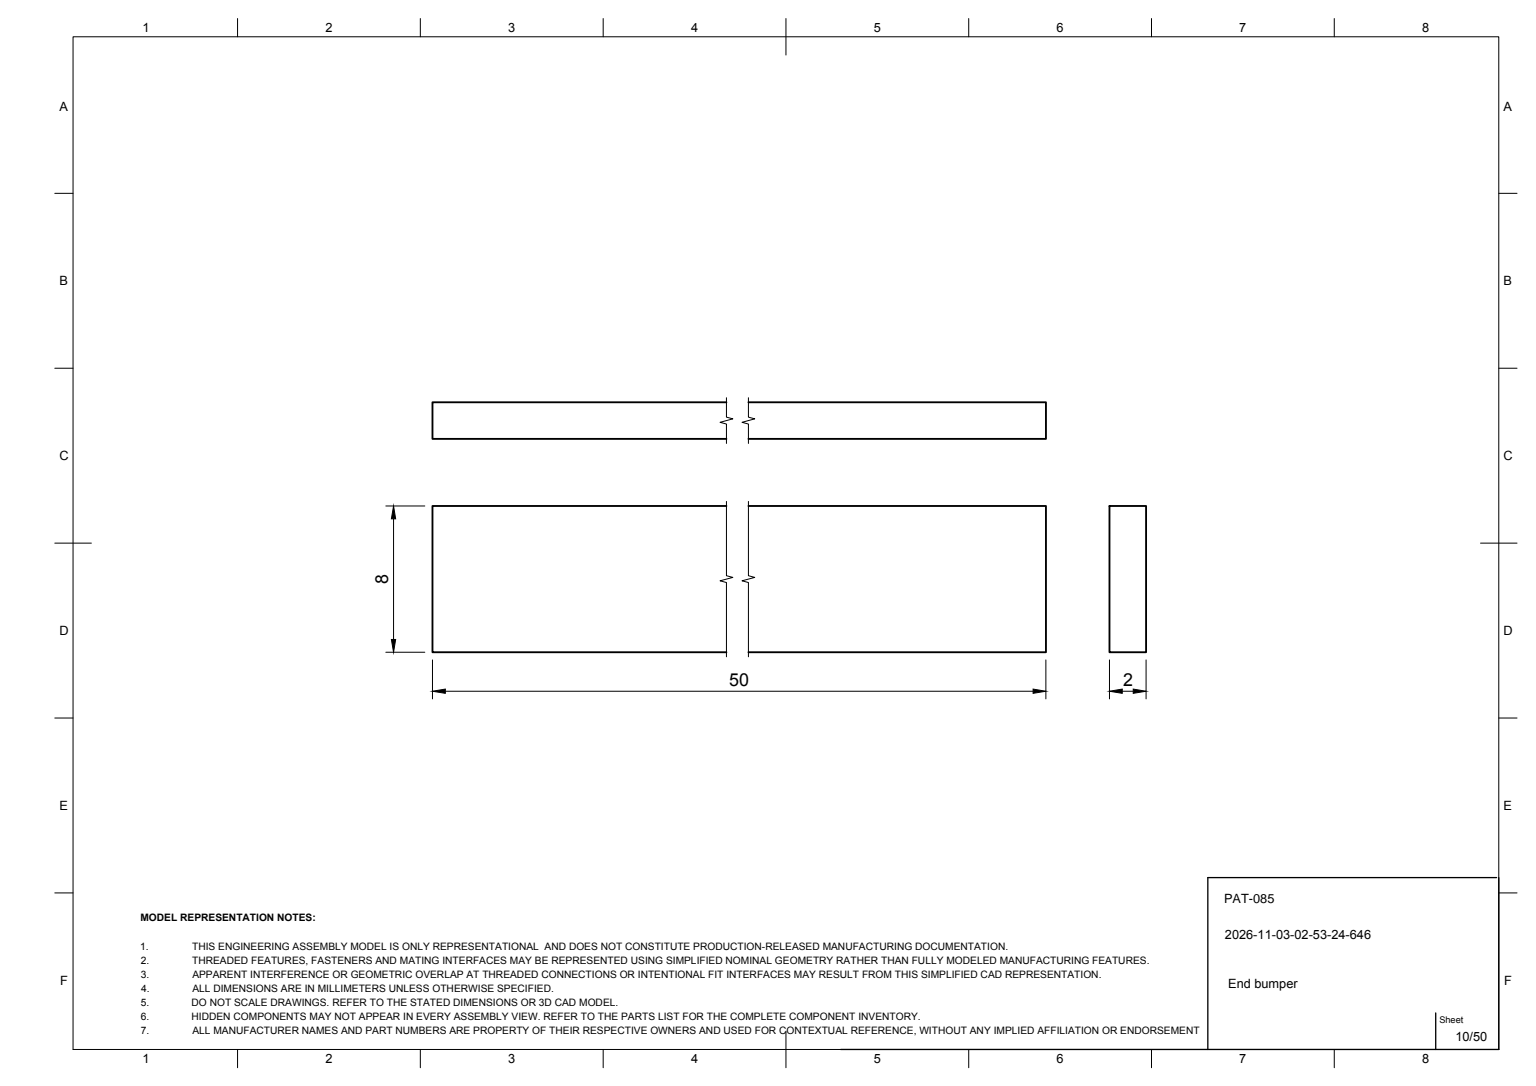
ISO-10303-21;
HEADER;
/* Generated by software containing ST-Developer
 * from STEP Tools, Inc. (www.steptools.com) 
 */

FILE_DESCRIPTION(
/* description */ ('Rack and pinion manual slide'),
/* implementation_level */ '2;1');

FILE_NAME(
/* name */ 'End bumper.step',
/* time_stamp */ '2026-10-28T03:22:49-07:00',
/* author */ (''),
/* organization */ (''),
/* preprocessor_version */ 'ST-DEVELOPER v20.2',
/* originating_system */ 'Autodesk Translation Framework v15.17.0.0',
/* authorisation */ '');

FILE_SCHEMA (('AUTOMOTIVE_DESIGN { 1 0 10303 214 3 1 1 }'));
ENDSEC;

DATA;
#10=MECHANICAL_DESIGN_GEOMETRIC_PRESENTATION_REPRESENTATION('',(#737),#34851);
#645=SHAPE_REPRESENTATION_RELATIONSHIP('SRR','None',#35080,#691);
#691=ADVANCED_BREP_SHAPE_REPRESENTATION('',(#790),#34805);
#737=STYLED_ITEM('',(#35404),#790);
#790=MANIFOLD_SOLID_BREP('Body1',#13757);
#1076=PLANE('',#14429);
#1077=PLANE('',#14430);
#1078=PLANE('',#14431);
#1079=PLANE('',#14432);
#1080=PLANE('',#14433);
#1081=PLANE('',#14434);
#1591=FACE_OUTER_BOUND('',#2376,.T.);
#1592=FACE_OUTER_BOUND('',#2377,.T.);
#1593=FACE_OUTER_BOUND('',#2378,.T.);
#1594=FACE_OUTER_BOUND('',#2379,.T.);
#1595=FACE_OUTER_BOUND('',#2380,.T.);
#1596=FACE_OUTER_BOUND('',#2381,.T.);
#2376=EDGE_LOOP('',(#9498,#9499,#9500,#9501));
#2377=EDGE_LOOP('',(#9502,#9503,#9504,#9505));
#2378=EDGE_LOOP('',(#9506,#9507,#9508,#9509));
#2379=EDGE_LOOP('',(#9510,#9511,#9512,#9513));
#2380=EDGE_LOOP('',(#9514,#9515,#9516,#9517));
#2381=EDGE_LOOP('',(#9518,#9519,#9520,#9521));
#3308=LINE('',#19744,#4599);
#3309=LINE('',#19746,#4600);
#3310=LINE('',#19748,#4601);
#3311=LINE('',#19749,#4602);
#3312=LINE('',#19752,#4603);
#3313=LINE('',#19754,#4604);
#3314=LINE('',#19755,#4605);
#3315=LINE('',#19758,#4606);
#3316=LINE('',#19760,#4607);
#3317=LINE('',#19761,#4608);
#3318=LINE('',#19763,#4609);
#3319=LINE('',#19764,#4610);
#4599=VECTOR('',#15910,1.);
#4600=VECTOR('',#15911,1.);
#4601=VECTOR('',#15912,1.);
#4602=VECTOR('',#15913,1.);
#4603=VECTOR('',#15916,1.);
#4604=VECTOR('',#15917,1.);
#4605=VECTOR('',#15918,1.);
#4606=VECTOR('',#15921,1.);
#4607=VECTOR('',#15922,1.);
#4608=VECTOR('',#15923,1.);
#4609=VECTOR('',#15926,1.);
#4610=VECTOR('',#15927,1.);
#6312=VERTEX_POINT('',#19742);
#6313=VERTEX_POINT('',#19743);
#6314=VERTEX_POINT('',#19745);
#6315=VERTEX_POINT('',#19747);
#6316=VERTEX_POINT('',#19751);
#6317=VERTEX_POINT('',#19753);
#6318=VERTEX_POINT('',#19757);
#6319=VERTEX_POINT('',#19759);
#7561=EDGE_CURVE('',#6312,#6313,#3308,.T.);
#7562=EDGE_CURVE('',#6313,#6314,#3309,.T.);
#7563=EDGE_CURVE('',#6315,#6314,#3310,.T.);
#7564=EDGE_CURVE('',#6312,#6315,#3311,.T.);
#7565=EDGE_CURVE('',#6316,#6312,#3312,.T.);
#7566=EDGE_CURVE('',#6317,#6315,#3313,.T.);
#7567=EDGE_CURVE('',#6316,#6317,#3314,.T.);
#7568=EDGE_CURVE('',#6318,#6316,#3315,.T.);
#7569=EDGE_CURVE('',#6319,#6317,#3316,.T.);
#7570=EDGE_CURVE('',#6318,#6319,#3317,.T.);
#7571=EDGE_CURVE('',#6313,#6318,#3318,.T.);
#7572=EDGE_CURVE('',#6314,#6319,#3319,.T.);
#9498=ORIENTED_EDGE('',*,*,#7561,.T.);
#9499=ORIENTED_EDGE('',*,*,#7562,.T.);
#9500=ORIENTED_EDGE('',*,*,#7563,.F.);
#9501=ORIENTED_EDGE('',*,*,#7564,.F.);
#9502=ORIENTED_EDGE('',*,*,#7565,.T.);
#9503=ORIENTED_EDGE('',*,*,#7564,.T.);
#9504=ORIENTED_EDGE('',*,*,#7566,.F.);
#9505=ORIENTED_EDGE('',*,*,#7567,.F.);
#9506=ORIENTED_EDGE('',*,*,#7568,.T.);
#9507=ORIENTED_EDGE('',*,*,#7567,.T.);
#9508=ORIENTED_EDGE('',*,*,#7569,.F.);
#9509=ORIENTED_EDGE('',*,*,#7570,.F.);
#9510=ORIENTED_EDGE('',*,*,#7571,.T.);
#9511=ORIENTED_EDGE('',*,*,#7570,.T.);
#9512=ORIENTED_EDGE('',*,*,#7572,.F.);
#9513=ORIENTED_EDGE('',*,*,#7562,.F.);
#9514=ORIENTED_EDGE('',*,*,#7572,.T.);
#9515=ORIENTED_EDGE('',*,*,#7569,.T.);
#9516=ORIENTED_EDGE('',*,*,#7566,.T.);
#9517=ORIENTED_EDGE('',*,*,#7563,.T.);
#9518=ORIENTED_EDGE('',*,*,#7571,.F.);
#9519=ORIENTED_EDGE('',*,*,#7561,.F.);
#9520=ORIENTED_EDGE('',*,*,#7565,.F.);
#9521=ORIENTED_EDGE('',*,*,#7568,.F.);
#13069=ADVANCED_FACE('',(#1591),#1076,.T.);
#13070=ADVANCED_FACE('',(#1592),#1077,.T.);
#13071=ADVANCED_FACE('',(#1593),#1078,.T.);
#13072=ADVANCED_FACE('',(#1594),#1079,.T.);
#13073=ADVANCED_FACE('',(#1595),#1080,.T.);
#13074=ADVANCED_FACE('',(#1596),#1081,.F.);
#13757=CLOSED_SHELL('',(#13069,#13070,#13071,#13072,#13073,#13074));
#14428=AXIS2_PLACEMENT_3D('',#19740,#15906,#15907);
#14429=AXIS2_PLACEMENT_3D('',#19741,#15908,#15909);
#14430=AXIS2_PLACEMENT_3D('',#19750,#15914,#15915);
#14431=AXIS2_PLACEMENT_3D('',#19756,#15919,#15920);
#14432=AXIS2_PLACEMENT_3D('',#19762,#15924,#15925);
#14433=AXIS2_PLACEMENT_3D('',#19765,#15928,#15929);
#14434=AXIS2_PLACEMENT_3D('',#19766,#15930,#15931);
#15906=DIRECTION('axis',(0.,0.,1.));
#15907=DIRECTION('refdir',(1.,0.,0.));
#15908=DIRECTION('center_axis',(0.,1.,0.));
#15909=DIRECTION('ref_axis',(-1.,0.,0.));
#15910=DIRECTION('',(-1.,0.,0.));
#15911=DIRECTION('',(0.,0.,1.));
#15912=DIRECTION('',(-1.,0.,0.));
#15913=DIRECTION('',(0.,0.,1.));
#15914=DIRECTION('center_axis',(1.,0.,0.));
#15915=DIRECTION('ref_axis',(0.,1.,0.));
#15916=DIRECTION('',(0.,1.,0.));
#15917=DIRECTION('',(0.,1.,0.));
#15918=DIRECTION('',(0.,0.,1.));
#15919=DIRECTION('center_axis',(0.,-1.,0.));
#15920=DIRECTION('ref_axis',(1.,0.,0.));
#15921=DIRECTION('',(1.,0.,0.));
#15922=DIRECTION('',(1.,0.,0.));
#15923=DIRECTION('',(0.,0.,1.));
#15924=DIRECTION('center_axis',(-1.,0.,0.));
#15925=DIRECTION('ref_axis',(0.,-1.,0.));
#15926=DIRECTION('',(0.,-1.,0.));
#15927=DIRECTION('',(0.,-1.,0.));
#15928=DIRECTION('center_axis',(0.,0.,1.));
#15929=DIRECTION('ref_axis',(1.,0.,0.));
#15930=DIRECTION('center_axis',(0.,0.,1.));
#15931=DIRECTION('ref_axis',(1.,0.,0.));
#19740=CARTESIAN_POINT('',(0.,0.,0.));
#19741=CARTESIAN_POINT('Origin',(-3.,2.5,6.2));
#19742=CARTESIAN_POINT('',(-3.,2.5,6.2));
#19743=CARTESIAN_POINT('',(-3.2,2.5,6.2));
#19744=CARTESIAN_POINT('',(-3.,2.5,6.2));
#19745=CARTESIAN_POINT('',(-3.2,2.5,7.));
#19746=CARTESIAN_POINT('',(-3.2,2.5,6.2));
#19747=CARTESIAN_POINT('',(-3.,2.5,7.));
#19748=CARTESIAN_POINT('',(-3.,2.5,7.));
#19749=CARTESIAN_POINT('',(-3.,2.5,6.2));
#19750=CARTESIAN_POINT('Origin',(-3.,-2.5,6.2));
#19751=CARTESIAN_POINT('',(-3.,-2.5,6.2));
#19752=CARTESIAN_POINT('',(-3.,-2.5,6.2));
#19753=CARTESIAN_POINT('',(-3.,-2.5,7.));
#19754=CARTESIAN_POINT('',(-3.,-2.5,7.));
#19755=CARTESIAN_POINT('',(-3.,-2.5,6.2));
#19756=CARTESIAN_POINT('Origin',(-3.2,-2.5,6.2));
#19757=CARTESIAN_POINT('',(-3.2,-2.5,6.2));
#19758=CARTESIAN_POINT('',(-3.2,-2.5,6.2));
#19759=CARTESIAN_POINT('',(-3.2,-2.5,7.));
#19760=CARTESIAN_POINT('',(-3.2,-2.5,7.));
#19761=CARTESIAN_POINT('',(-3.2,-2.5,6.2));
#19762=CARTESIAN_POINT('Origin',(-3.2,2.5,6.2));
#19763=CARTESIAN_POINT('',(-3.2,2.5,6.2));
#19764=CARTESIAN_POINT('',(-3.2,2.5,7.));
#19765=CARTESIAN_POINT('Origin',(-3.1,0.,7.));
#19766=CARTESIAN_POINT('Origin',(-3.1,0.,6.2));
#34751=UNCERTAINTY_MEASURE_WITH_UNIT(LENGTH_MEASURE(0.001),#34852,
'DISTANCE_ACCURACY_VALUE',
'Maximum model space distance between geometric entities at asserted c
onnectivities');
#34797=UNCERTAINTY_MEASURE_WITH_UNIT(LENGTH_MEASURE(0.001),#34852,
'DISTANCE_ACCURACY_VALUE',
'Maximum model space distance between geometric entities at asserted c
onnectivities');
#34805=(
GEOMETRIC_REPRESENTATION_CONTEXT(3)
GLOBAL_UNCERTAINTY_ASSIGNED_CONTEXT((#34751))
GLOBAL_UNIT_ASSIGNED_CONTEXT((#34852,#34854,#34855))
REPRESENTATION_CONTEXT('','3D')
);
#34851=(
GEOMETRIC_REPRESENTATION_CONTEXT(3)
GLOBAL_UNCERTAINTY_ASSIGNED_CONTEXT((#34797))
GLOBAL_UNIT_ASSIGNED_CONTEXT((#34852,#34854,#34855))
REPRESENTATION_CONTEXT('','3D')
);
#34852=(
LENGTH_UNIT()
NAMED_UNIT(*)
SI_UNIT(.CENTI.,.METRE.)
);
#34854=(
NAMED_UNIT(*)
PLANE_ANGLE_UNIT()
SI_UNIT($,.RADIAN.)
);
#34855=(
NAMED_UNIT(*)
SI_UNIT($,.STERADIAN.)
SOLID_ANGLE_UNIT()
);
#34863=SHAPE_DEFINITION_REPRESENTATION(#34916,#35080);
#34916=PRODUCT_DEFINITION_SHAPE('',$,#35134);
#35080=SHAPE_REPRESENTATION('',(#14428),#34805);
#35126=PRODUCT_DEFINITION_CONTEXT('part definition',#35287,'design');
#35134=PRODUCT_DEFINITION('End bumper','End bumper',#35187,#35126);
#35187=PRODUCT_DEFINITION_FORMATION('',$,#35296);
#35287=APPLICATION_CONTEXT(
'Core Data for Automotive Mechanical Design Process');
#35288=PRODUCT_CONTEXT('part definition',#35287,'mechanical');
#35296=PRODUCT('End bumper','End bumper','End bumper',(#35288));
#35398=COLOUR_RGB('Sky Blue',0.24,0.69,0.87);
#35399=FILL_AREA_STYLE_COLOUR('',#35398);
#35400=FILL_AREA_STYLE('',(#35399));
#35401=SURFACE_STYLE_FILL_AREA(#35400);
#35402=SURFACE_SIDE_STYLE('',(#35401));
#35403=SURFACE_STYLE_USAGE(.BOTH.,#35402);
#35404=PRESENTATION_STYLE_ASSIGNMENT((#35403));
ENDSEC;
END-ISO-10303-21;
